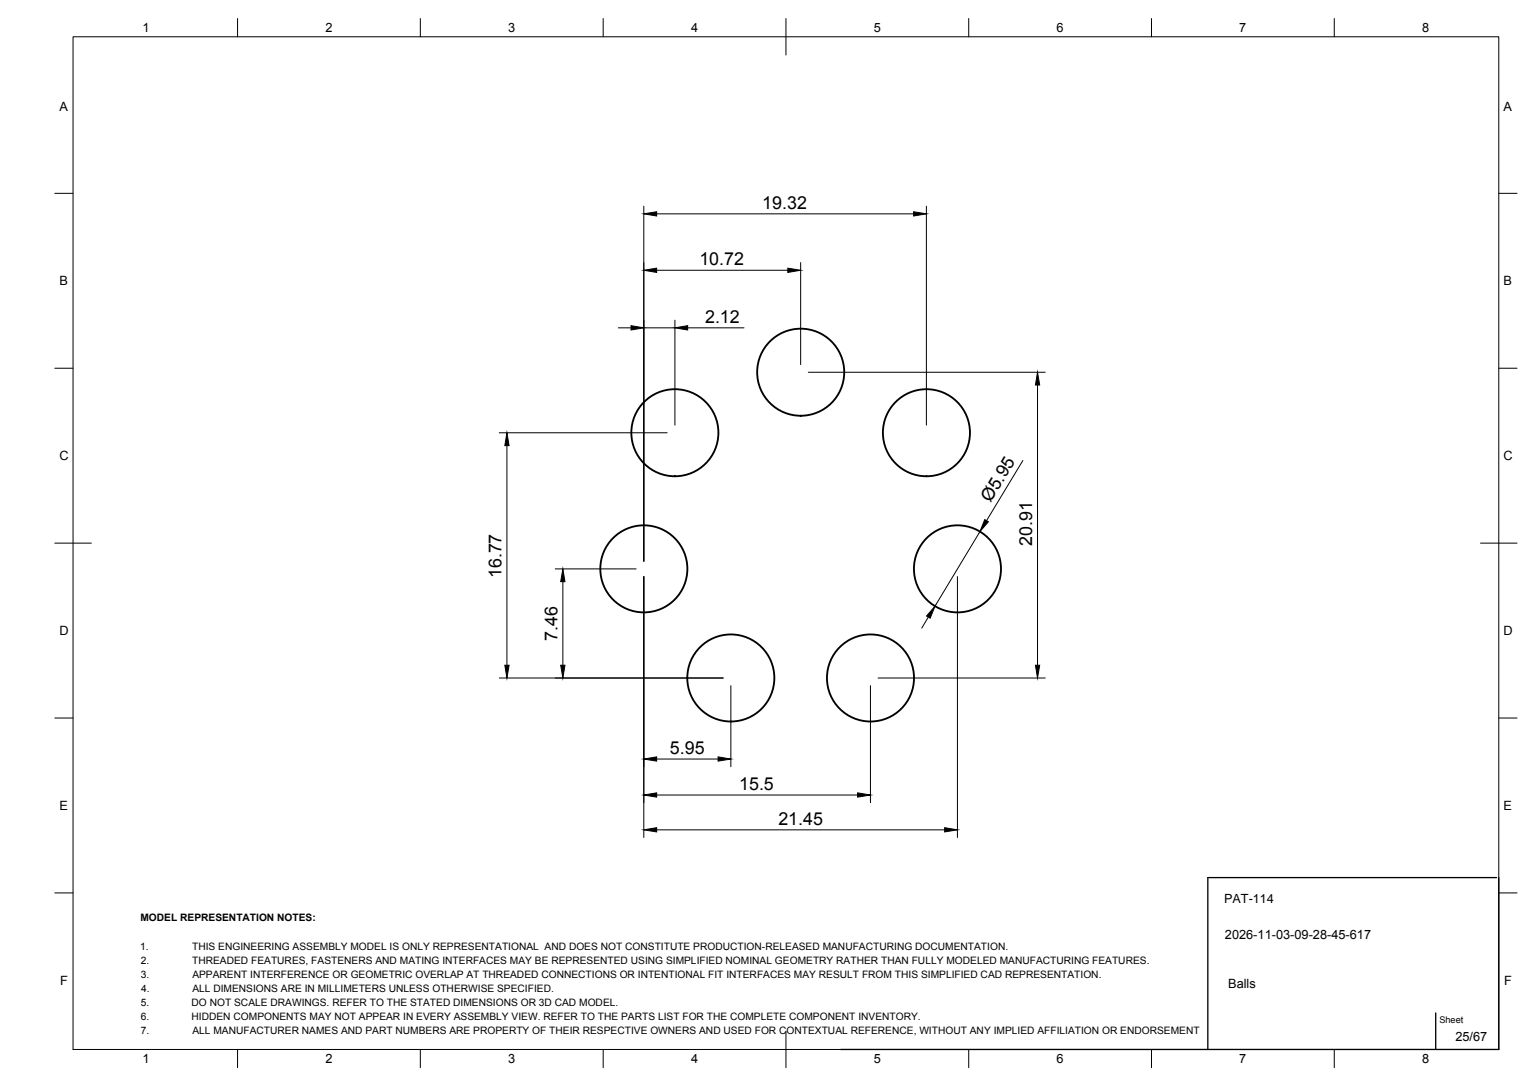
ISO-10303-21;
HEADER;
/* Generated by software containing ST-Developer
 * from STEP Tools, Inc. (www.steptools.com) 
 */

FILE_DESCRIPTION(
/* description */ ('Two-stage gear reducer in split housing'),
/* implementation_level */ '2;1');

FILE_NAME(
/* name */ 'Balls.step',
/* time_stamp */ '2026-10-28T03:22:31-07:00',
/* author */ (''),
/* organization */ (''),
/* preprocessor_version */ 'ST-DEVELOPER v20.2',
/* originating_system */ 'Autodesk Translation Framework v15.17.0.0',
/* authorisation */ '');

FILE_SCHEMA (('AUTOMOTIVE_DESIGN { 1 0 10303 214 3 1 1 }'));
ENDSEC;

DATA;
#10=MECHANICAL_DESIGN_GEOMETRIC_PRESENTATION_REPRESENTATION('',(#1253,#1254,#1255,#1256,#1257,#1258,#1259),#73366);
#1067=SPHERICAL_SURFACE('',#17458,0.29765);
#1068=SPHERICAL_SURFACE('',#17460,0.29765);
#1069=SPHERICAL_SURFACE('',#17462,0.29765);
#1070=SPHERICAL_SURFACE('',#17464,0.29765);
#1071=SPHERICAL_SURFACE('',#17466,0.29765);
#1072=SPHERICAL_SURFACE('',#17468,0.29765);
#1073=SPHERICAL_SURFACE('',#17470,0.29765);
#1141=SHAPE_REPRESENTATION_RELATIONSHIP('SRR','None',#73629,#1197);
#1197=ADVANCED_BREP_SHAPE_REPRESENTATION('',(#1323,#1324,#1325,#1326,#1327,
#1328,#1329),#73325);
#1253=STYLED_ITEM('',(#73988),#1323);
#1254=STYLED_ITEM('',(#73988),#1324);
#1255=STYLED_ITEM('',(#73988),#1325);
#1256=STYLED_ITEM('',(#73988),#1326);
#1257=STYLED_ITEM('',(#73988),#1327);
#1258=STYLED_ITEM('',(#73988),#1328);
#1259=STYLED_ITEM('',(#73988),#1329);
#1323=MANIFOLD_SOLID_BREP('Body1',#16142);
#1324=MANIFOLD_SOLID_BREP('Body2',#16143);
#1325=MANIFOLD_SOLID_BREP('Body3',#16144);
#1326=MANIFOLD_SOLID_BREP('Body4',#16145);
#1327=MANIFOLD_SOLID_BREP('Body5',#16146);
#1328=MANIFOLD_SOLID_BREP('Body6',#16147);
#1329=MANIFOLD_SOLID_BREP('Body7',#16148);
#2316=FACE_OUTER_BOUND('',#3378,.T.);
#2317=FACE_OUTER_BOUND('',#3379,.T.);
#2318=FACE_OUTER_BOUND('',#3380,.T.);
#2319=FACE_OUTER_BOUND('',#3381,.T.);
#2320=FACE_OUTER_BOUND('',#3382,.T.);
#2321=FACE_OUTER_BOUND('',#3383,.T.);
#2322=FACE_OUTER_BOUND('',#3384,.T.);
#3378=EDGE_LOOP('',(#11879,#11880));
#3379=EDGE_LOOP('',(#11881,#11882));
#3380=EDGE_LOOP('',(#11883,#11884));
#3381=EDGE_LOOP('',(#11885,#11886));
#3382=EDGE_LOOP('',(#11887,#11888));
#3383=EDGE_LOOP('',(#11889,#11890));
#3384=EDGE_LOOP('',(#11891,#11892));
#6413=CIRCLE('',#17459,0.29765);
#6414=CIRCLE('',#17461,0.29765);
#6415=CIRCLE('',#17463,0.29765);
#6416=CIRCLE('',#17465,0.29765);
#6417=CIRCLE('',#17467,0.29765);
#6418=CIRCLE('',#17469,0.29765);
#6419=CIRCLE('',#17471,0.29765);
#7279=VERTEX_POINT('',#24253);
#7280=VERTEX_POINT('',#24254);
#7281=VERTEX_POINT('',#24257);
#7282=VERTEX_POINT('',#24258);
#7283=VERTEX_POINT('',#24261);
#7284=VERTEX_POINT('',#24262);
#7285=VERTEX_POINT('',#24265);
#7286=VERTEX_POINT('',#24266);
#7287=VERTEX_POINT('',#24269);
#7288=VERTEX_POINT('',#24270);
#7289=VERTEX_POINT('',#24273);
#7290=VERTEX_POINT('',#24274);
#7291=VERTEX_POINT('',#24277);
#7292=VERTEX_POINT('',#24278);
#8993=EDGE_CURVE('',#7279,#7280,#6413,.T.);
#8994=EDGE_CURVE('',#7281,#7282,#6414,.T.);
#8995=EDGE_CURVE('',#7283,#7284,#6415,.T.);
#8996=EDGE_CURVE('',#7285,#7286,#6416,.T.);
#8997=EDGE_CURVE('',#7287,#7288,#6417,.T.);
#8998=EDGE_CURVE('',#7289,#7290,#6418,.T.);
#8999=EDGE_CURVE('',#7291,#7292,#6419,.T.);
#11879=ORIENTED_EDGE('',*,*,#8993,.T.);
#11880=ORIENTED_EDGE('',*,*,#8993,.F.);
#11881=ORIENTED_EDGE('',*,*,#8994,.T.);
#11882=ORIENTED_EDGE('',*,*,#8994,.F.);
#11883=ORIENTED_EDGE('',*,*,#8995,.T.);
#11884=ORIENTED_EDGE('',*,*,#8995,.F.);
#11885=ORIENTED_EDGE('',*,*,#8996,.T.);
#11886=ORIENTED_EDGE('',*,*,#8996,.F.);
#11887=ORIENTED_EDGE('',*,*,#8997,.T.);
#11888=ORIENTED_EDGE('',*,*,#8997,.F.);
#11889=ORIENTED_EDGE('',*,*,#8998,.T.);
#11890=ORIENTED_EDGE('',*,*,#8998,.F.);
#11891=ORIENTED_EDGE('',*,*,#8999,.T.);
#11892=ORIENTED_EDGE('',*,*,#8999,.F.);
#15523=ADVANCED_FACE('',(#2316),#1067,.T.);
#15524=ADVANCED_FACE('',(#2317),#1068,.T.);
#15525=ADVANCED_FACE('',(#2318),#1069,.T.);
#15526=ADVANCED_FACE('',(#2319),#1070,.T.);
#15527=ADVANCED_FACE('',(#2320),#1071,.T.);
#15528=ADVANCED_FACE('',(#2321),#1072,.T.);
#15529=ADVANCED_FACE('',(#2322),#1073,.T.);
#16142=CLOSED_SHELL('',(#15523));
#16143=CLOSED_SHELL('',(#15524));
#16144=CLOSED_SHELL('',(#15525));
#16145=CLOSED_SHELL('',(#15526));
#16146=CLOSED_SHELL('',(#15527));
#16147=CLOSED_SHELL('',(#15528));
#16148=CLOSED_SHELL('',(#15529));
#17457=AXIS2_PLACEMENT_3D('',#24251,#20125,#20126);
#17458=AXIS2_PLACEMENT_3D('',#24252,#20127,#20128);
#17459=AXIS2_PLACEMENT_3D('',#24255,#20129,#20130);
#17460=AXIS2_PLACEMENT_3D('',#24256,#20131,#20132);
#17461=AXIS2_PLACEMENT_3D('',#24259,#20133,#20134);
#17462=AXIS2_PLACEMENT_3D('',#24260,#20135,#20136);
#17463=AXIS2_PLACEMENT_3D('',#24263,#20137,#20138);
#17464=AXIS2_PLACEMENT_3D('',#24264,#20139,#20140);
#17465=AXIS2_PLACEMENT_3D('',#24267,#20141,#20142);
#17466=AXIS2_PLACEMENT_3D('',#24268,#20143,#20144);
#17467=AXIS2_PLACEMENT_3D('',#24271,#20145,#20146);
#17468=AXIS2_PLACEMENT_3D('',#24272,#20147,#20148);
#17469=AXIS2_PLACEMENT_3D('',#24275,#20149,#20150);
#17470=AXIS2_PLACEMENT_3D('',#24276,#20151,#20152);
#17471=AXIS2_PLACEMENT_3D('',#24279,#20153,#20154);
#20125=DIRECTION('axis',(0.,0.,1.));
#20126=DIRECTION('refdir',(1.,0.,0.));
#20127=DIRECTION('center_axis',(0.,0.,1.));
#20128=DIRECTION('ref_axis',(1.,0.,0.));
#20129=DIRECTION('center_axis',(1.22464679914735E-16,-1.,0.));
#20130=DIRECTION('ref_axis',(-1.,-1.22464679914735E-16,0.));
#20131=DIRECTION('center_axis',(0.78183148246803,0.,0.623489801858733));
#20132=DIRECTION('ref_axis',(0.623489801858734,0.,-0.78183148246803));
#20133=DIRECTION('center_axis',(7.63554790147315E-17,-1.,-9.57467422477103E-17));
#20134=DIRECTION('ref_axis',(-0.623489801858734,-1.22464679914735E-16,0.78183148246803));
#20135=DIRECTION('center_axis',(0.974927912181824,0.,-0.222520933956314));
#20136=DIRECTION('ref_axis',(-0.222520933956314,0.,-0.974927912181824));
#20137=DIRECTION('center_axis',(-2.7250954951288E-17,-1.,-1.19394234705288E-16));
#20138=DIRECTION('ref_axis',(0.222520933956314,-1.22464679914735E-16,0.974927912181824));
#20139=DIRECTION('center_axis',(0.433883739117558,0.,-0.900968867902419));
#20140=DIRECTION('ref_axis',(-0.900968867902419,0.,-0.433883739117558));
#20141=DIRECTION('center_axis',(-1.10336864020811E-16,-1.,-5.31354332312403E-17));
#20142=DIRECTION('ref_axis',(0.900968867902419,-1.22464679914735E-16,0.433883739117558));
#20143=DIRECTION('center_axis',(-0.433883739117558,0.,-0.900968867902419));
#20144=DIRECTION('ref_axis',(-0.900968867902419,0.,0.433883739117558));
#20145=DIRECTION('center_axis',(-1.10336864020811E-16,-1.,5.31354332312403E-17));
#20146=DIRECTION('ref_axis',(0.900968867902419,-1.22464679914735E-16,-0.433883739117558));
#20147=DIRECTION('center_axis',(-0.974927912181824,0.,-0.222520933956314));
#20148=DIRECTION('ref_axis',(-0.222520933956315,0.,0.974927912181824));
#20149=DIRECTION('center_axis',(-2.7250954951288E-17,-1.,1.19394234705288E-16));
#20150=DIRECTION('ref_axis',(0.222520933956315,-1.22464679914735E-16,-0.974927912181824));
#20151=DIRECTION('center_axis',(-0.78183148246803,0.,0.623489801858734));
#20152=DIRECTION('ref_axis',(0.623489801858733,0.,0.78183148246803));
#20153=DIRECTION('center_axis',(7.63554790147315E-17,-1.,9.57467422477103E-17));
#20154=DIRECTION('ref_axis',(-0.623489801858733,-1.22464679914735E-16,-0.78183148246803));
#24251=CARTESIAN_POINT('',(0.,0.,0.));
#24252=CARTESIAN_POINT('Origin',(1.1,0.,0.));
#24253=CARTESIAN_POINT('',(1.1,-2.23201749654651E-33,0.29765));
#24254=CARTESIAN_POINT('',(1.1,-2.23201749654651E-33,-0.29765));
#24255=CARTESIAN_POINT('Origin',(1.1,0.,0.));
#24256=CARTESIAN_POINT('Origin',(0.685838782044607,0.,-0.860014630714833));
#24257=CARTESIAN_POINT('',(0.918550922801216,-5.31350540756609E-33,-0.674432891191581));
#24258=CARTESIAN_POINT('',(0.453126641287998,8.49470414473068E-34,-1.04559637023808));
#24259=CARTESIAN_POINT('Origin',(0.685838782044607,0.,-0.860014630714833));
#24260=CARTESIAN_POINT('Origin',(-0.244773027351946,0.,-1.07242070340001));
#24261=CARTESIAN_POINT('',(0.0454142657089739,-2.23201749654651E-33,-1.1386540593921));
#24262=CARTESIAN_POINT('',(-0.534960320412865,-2.23201749654651E-33,-1.00618734740791));
#24263=CARTESIAN_POINT('Origin',(-0.244773027351946,0.,-1.07242070340001));
#24264=CARTESIAN_POINT('Origin',(-0.991065754692661,0.,-0.477272113029314));
#24265=CARTESIAN_POINT('',(-0.86192025974432,8.49470414473067E-34,-0.745445496560469));
#24266=CARTESIAN_POINT('',(-1.120211249641,-5.31350540756609E-33,-0.209098729498159));
#24267=CARTESIAN_POINT('Origin',(-0.991065754692661,0.,-0.477272113029314));
#24268=CARTESIAN_POINT('Origin',(-0.991065754692661,0.,0.477272113029314));
#24269=CARTESIAN_POINT('',(-1.120211249641,-2.23201749654651E-33,0.209098729498159));
#24270=CARTESIAN_POINT('',(-0.86192025974432,-2.23201749654651E-33,0.745445496560469));
#24271=CARTESIAN_POINT('Origin',(-0.991065754692661,0.,0.477272113029314));
#24272=CARTESIAN_POINT('Origin',(-0.244773027351946,0.,1.07242070340001));
#24273=CARTESIAN_POINT('',(-0.534960320412866,-2.23201749654651E-33,1.00618734740791));
#24274=CARTESIAN_POINT('',(0.0454142657089737,-2.23201749654651E-33,1.1386540593921));
#24275=CARTESIAN_POINT('Origin',(-0.244773027351946,0.,1.07242070340001));
#24276=CARTESIAN_POINT('Origin',(0.685838782044607,0.,0.860014630714833));
#24277=CARTESIAN_POINT('',(0.453126641287998,-2.23201749654651E-33,1.04559637023808));
#24278=CARTESIAN_POINT('',(0.918550922801216,-2.23201749654651E-33,0.674432891191581));
#24279=CARTESIAN_POINT('Origin',(0.685838782044607,0.,0.860014630714833));
#73261=UNCERTAINTY_MEASURE_WITH_UNIT(LENGTH_MEASURE(0.001),#73367,
'DISTANCE_ACCURACY_VALUE',
'Maximum model space distance between geometric entities at asserted c
onnectivities');
#73302=UNCERTAINTY_MEASURE_WITH_UNIT(LENGTH_MEASURE(0.001),#73367,
'DISTANCE_ACCURACY_VALUE',
'Maximum model space distance between geometric entities at asserted c
onnectivities');
#73325=(
GEOMETRIC_REPRESENTATION_CONTEXT(3)
GLOBAL_UNCERTAINTY_ASSIGNED_CONTEXT((#73261))
GLOBAL_UNIT_ASSIGNED_CONTEXT((#73367,#73369,#73370))
REPRESENTATION_CONTEXT('','3D')
);
#73366=(
GEOMETRIC_REPRESENTATION_CONTEXT(3)
GLOBAL_UNCERTAINTY_ASSIGNED_CONTEXT((#73302))
GLOBAL_UNIT_ASSIGNED_CONTEXT((#73367,#73369,#73370))
REPRESENTATION_CONTEXT('','3D')
);
#73367=(
LENGTH_UNIT()
NAMED_UNIT(*)
SI_UNIT(.CENTI.,.METRE.)
);
#73369=(
NAMED_UNIT(*)
PLANE_ANGLE_UNIT()
SI_UNIT($,.RADIAN.)
);
#73370=(
NAMED_UNIT(*)
SI_UNIT($,.STERADIAN.)
SOLID_ANGLE_UNIT()
);
#73393=SHAPE_DEFINITION_REPRESENTATION(#73456,#73629);
#73456=PRODUCT_DEFINITION_SHAPE('',$,#73693);
#73629=SHAPE_REPRESENTATION('',(#17457),#73325);
#73670=PRODUCT_DEFINITION_CONTEXT('part definition',#73861,'design');
#73693=PRODUCT_DEFINITION('Balls','Balls',#73756,#73670);
#73756=PRODUCT_DEFINITION_FORMATION('',$,#73885);
#73861=APPLICATION_CONTEXT(
'Core Data for Automotive Mechanical Design Process');
#73862=PRODUCT_CONTEXT('part definition',#73861,'mechanical');
#73885=PRODUCT('Balls','Balls','Balls',(#73862));
#73982=COLOUR_RGB('Grey',0.48,0.52,0.57);
#73983=FILL_AREA_STYLE_COLOUR('',#73982);
#73984=FILL_AREA_STYLE('',(#73983));
#73985=SURFACE_STYLE_FILL_AREA(#73984);
#73986=SURFACE_SIDE_STYLE('',(#73985));
#73987=SURFACE_STYLE_USAGE(.BOTH.,#73986);
#73988=PRESENTATION_STYLE_ASSIGNMENT((#73987));
ENDSEC;
END-ISO-10303-21;
